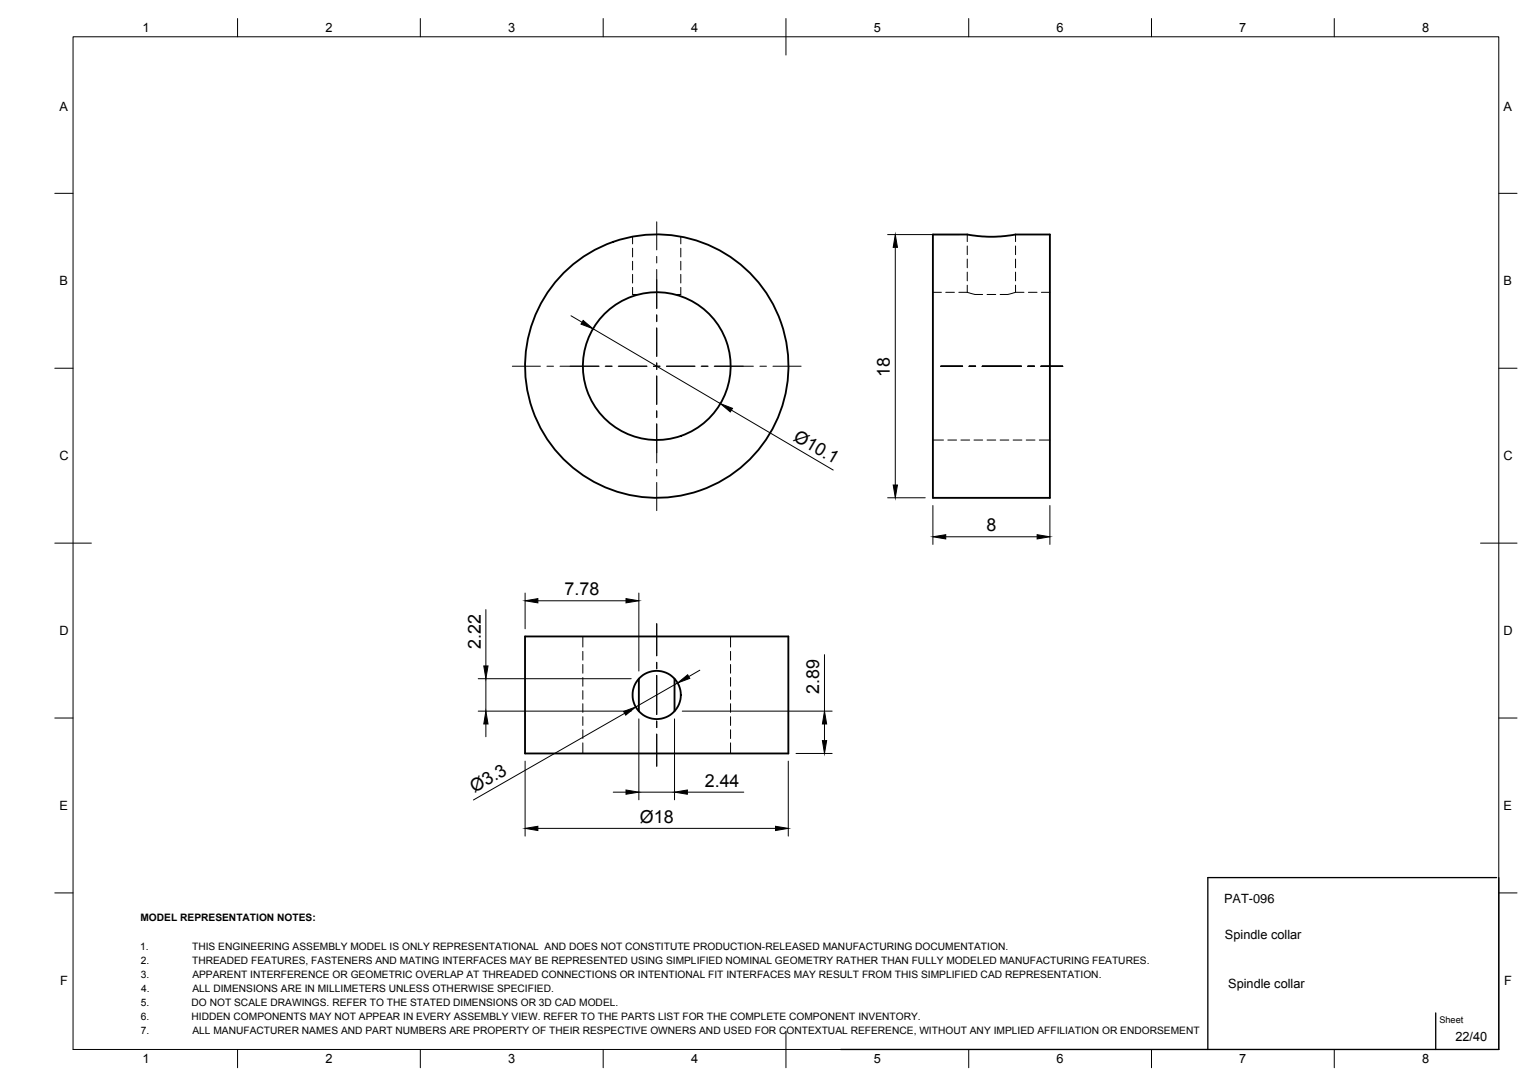
ISO-10303-21;
HEADER;
/* Generated by software containing ST-Developer
 * from STEP Tools, Inc. (www.steptools.com) 
 */

FILE_DESCRIPTION(
/* description */ ('PAT-096'),
/* implementation_level */ '2;1');

FILE_NAME(
/* name */ 'Spindle collar.step',
/* time_stamp */ '2026-10-29T17:03:14-07:00',
/* author */ (''),
/* organization */ (''),
/* preprocessor_version */ 'ST-DEVELOPER v20.2',
/* originating_system */ 'Autodesk Translation Framework v15.17.0.0',
/* authorisation */ '');

FILE_SCHEMA (('AUTOMOTIVE_DESIGN { 1 0 10303 214 3 1 1 }'));
ENDSEC;

DATA;
#10=MECHANICAL_DESIGN_GEOMETRIC_PRESENTATION_REPRESENTATION('',(#421),#10650);
#307=B_SPLINE_CURVE_WITH_KNOTS('',3,(#9836,#9837,#9838,#9839,#9840,#9841,
#9842,#9843,#9844,#9845,#9846,#9847,#9848,#9849),.UNSPECIFIED.,.F.,.F.,
(4,2,2,2,2,2,4),(0.618551524396293,0.626563103102765,0.689203386094988,
0.751843669087211,0.814483952079434,0.877124235071657,0.88513581377813),
 .UNSPECIFIED.);
#308=B_SPLINE_CURVE_WITH_KNOTS('',3,(#9853,#9854,#9855,#9856,#9857,#9858,
#9859,#9860),.UNSPECIFIED.,.F.,.F.,(4,2,2,4),(0.250614556362404,0.313254839354627,
0.37589512234685,0.383906701053323),.UNSPECIFIED.);
#309=B_SPLINE_CURVE_WITH_KNOTS('',3,(#9864,#9865,#9866,#9867,#9868,#9869,
#9870,#9871,#9872,#9873,#9874,#9875,#9876,#9877,#9878,#9879,#9880,#9881,
#9882,#9883,#9884,#9885,#9886,#9887,#9888,#9889),.UNSPECIFIED.,.F.,.F.,
(4,2,2,2,2,2,2,2,2,2,2,2,4),(0.,0.0623062782223143,0.124612556444629,0.186916384615149,
0.249220212785669,0.31152404095619,0.37382786912671,0.436134147349024,0.498440425571339,
0.560746703793653,0.623052982015967,0.685356810186488,0.747660638357008),
 .UNSPECIFIED.);
#310=B_SPLINE_CURVE_WITH_KNOTS('',3,(#9890,#9891,#9892,#9893,#9894,#9895,
#9896,#9897,#9898,#9899),.UNSPECIFIED.,.F.,.F.,(4,2,2,2,4),(0.747660638357008,
0.809964466527528,0.872268294698049,0.934574572920363,0.996880851142677),
 .UNSPECIFIED.);
#311=B_SPLINE_CURVE_WITH_KNOTS('',3,(#9900,#9901,#9902,#9903,#9904,#9905,
#9906,#9907),.UNSPECIFIED.,.F.,.F.,(4,2,2,4),(0.117322411671485,0.125333990377958,
0.187974273370181,0.250614556362404),.UNSPECIFIED.);
#351=SHAPE_REPRESENTATION_RELATIONSHIP('SRR','None',#10813,#382);
#382=ADVANCED_BREP_SHAPE_REPRESENTATION('',(#459),#10631);
#421=STYLED_ITEM('',(#11057),#459);
#459=MANIFOLD_SOLID_BREP('Body1',#5555);
#553=FACE_BOUND('',#1400,.T.);
#554=FACE_BOUND('',#1402,.T.);
#555=FACE_BOUND('',#1404,.T.);
#556=FACE_BOUND('',#1406,.T.);
#701=PLANE('',#6337);
#702=PLANE('',#6341);
#703=PLANE('',#6348);
#704=PLANE('',#6349);
#980=FACE_OUTER_BOUND('',#1396,.T.);
#981=FACE_OUTER_BOUND('',#1397,.T.);
#982=FACE_OUTER_BOUND('',#1398,.T.);
#983=FACE_OUTER_BOUND('',#1399,.T.);
#984=FACE_OUTER_BOUND('',#1401,.T.);
#985=FACE_OUTER_BOUND('',#1403,.T.);
#986=FACE_OUTER_BOUND('',#1405,.T.);
#1396=EDGE_LOOP('',(#4517,#4518));
#1397=EDGE_LOOP('',(#4519,#4520,#4521,#4522,#4523,#4524,#4525,#4526,#4527));
#1398=EDGE_LOOP('',(#4528,#4529));
#1399=EDGE_LOOP('',(#4530,#4531,#4532,#4533));
#1400=EDGE_LOOP('',(#4534,#4535,#4536,#4537,#4538));
#1401=EDGE_LOOP('',(#4539,#4540,#4541,#4542));
#1402=EDGE_LOOP('',(#4543,#4544));
#1403=EDGE_LOOP('',(#4545));
#1404=EDGE_LOOP('',(#4546));
#1405=EDGE_LOOP('',(#4547));
#1406=EDGE_LOOP('',(#4548));
#1769=LINE('',#9832,#2098);
#1770=LINE('',#9862,#2099);
#1771=LINE('',#9909,#2100);
#1772=LINE('',#9914,#2101);
#1773=LINE('',#9920,#2102);
#2098=VECTOR('',#7685,1.);
#2099=VECTOR('',#7692,0.165);
#2100=VECTOR('',#7695,1.);
#2101=VECTOR('',#7700,0.505);
#2102=VECTOR('',#7707,0.9);
#2466=CIRCLE('',#6338,0.165);
#2467=CIRCLE('',#6340,0.165);
#2468=CIRCLE('',#6343,0.505);
#2469=CIRCLE('',#6344,0.505);
#2470=CIRCLE('',#6346,0.9);
#2471=CIRCLE('',#6347,0.9);
#2853=VERTEX_POINT('',#9830);
#2854=VERTEX_POINT('',#9831);
#2855=VERTEX_POINT('',#9835);
#2856=VERTEX_POINT('',#9850);
#2857=VERTEX_POINT('',#9852);
#2858=VERTEX_POINT('',#9861);
#2859=VERTEX_POINT('',#9863);
#2860=VERTEX_POINT('',#9911);
#2861=VERTEX_POINT('',#9913);
#2862=VERTEX_POINT('',#9917);
#2863=VERTEX_POINT('',#9919);
#3437=EDGE_CURVE('',#2853,#2854,#1769,.T.);
#3438=EDGE_CURVE('',#2853,#2854,#2466,.T.);
#3439=EDGE_CURVE('',#2855,#2853,#307,.T.);
#3440=EDGE_CURVE('',#2856,#2855,#2467,.T.);
#3441=EDGE_CURVE('',#2857,#2856,#308,.T.);
#3442=EDGE_CURVE('',#2857,#2858,#1770,.T.);
#3443=EDGE_CURVE('',#2859,#2858,#309,.T.);
#3444=EDGE_CURVE('',#2858,#2859,#310,.T.);
#3445=EDGE_CURVE('',#2854,#2857,#311,.T.);
#3446=EDGE_CURVE('',#2856,#2855,#1771,.T.);
#3447=EDGE_CURVE('',#2860,#2860,#2468,.T.);
#3448=EDGE_CURVE('',#2860,#2861,#1772,.T.);
#3449=EDGE_CURVE('',#2861,#2861,#2469,.T.);
#3450=EDGE_CURVE('',#2862,#2862,#2470,.T.);
#3451=EDGE_CURVE('',#2862,#2863,#1773,.T.);
#3452=EDGE_CURVE('',#2863,#2863,#2471,.T.);
#4517=ORIENTED_EDGE('',*,*,#3437,.F.);
#4518=ORIENTED_EDGE('',*,*,#3438,.T.);
#4519=ORIENTED_EDGE('',*,*,#3439,.F.);
#4520=ORIENTED_EDGE('',*,*,#3440,.F.);
#4521=ORIENTED_EDGE('',*,*,#3441,.F.);
#4522=ORIENTED_EDGE('',*,*,#3442,.T.);
#4523=ORIENTED_EDGE('',*,*,#3443,.F.);
#4524=ORIENTED_EDGE('',*,*,#3444,.F.);
#4525=ORIENTED_EDGE('',*,*,#3442,.F.);
#4526=ORIENTED_EDGE('',*,*,#3445,.F.);
#4527=ORIENTED_EDGE('',*,*,#3438,.F.);
#4528=ORIENTED_EDGE('',*,*,#3446,.F.);
#4529=ORIENTED_EDGE('',*,*,#3440,.T.);
#4530=ORIENTED_EDGE('',*,*,#3447,.F.);
#4531=ORIENTED_EDGE('',*,*,#3448,.T.);
#4532=ORIENTED_EDGE('',*,*,#3449,.T.);
#4533=ORIENTED_EDGE('',*,*,#3448,.F.);
#4534=ORIENTED_EDGE('',*,*,#3445,.T.);
#4535=ORIENTED_EDGE('',*,*,#3441,.T.);
#4536=ORIENTED_EDGE('',*,*,#3446,.T.);
#4537=ORIENTED_EDGE('',*,*,#3439,.T.);
#4538=ORIENTED_EDGE('',*,*,#3437,.T.);
#4539=ORIENTED_EDGE('',*,*,#3450,.F.);
#4540=ORIENTED_EDGE('',*,*,#3451,.T.);
#4541=ORIENTED_EDGE('',*,*,#3452,.T.);
#4542=ORIENTED_EDGE('',*,*,#3451,.F.);
#4543=ORIENTED_EDGE('',*,*,#3443,.T.);
#4544=ORIENTED_EDGE('',*,*,#3444,.T.);
#4545=ORIENTED_EDGE('',*,*,#3450,.T.);
#4546=ORIENTED_EDGE('',*,*,#3447,.T.);
#4547=ORIENTED_EDGE('',*,*,#3452,.F.);
#4548=ORIENTED_EDGE('',*,*,#3449,.F.);
#5146=CYLINDRICAL_SURFACE('',#6339,0.165);
#5147=CYLINDRICAL_SURFACE('',#6342,0.505);
#5148=CYLINDRICAL_SURFACE('',#6345,0.9);
#5385=ADVANCED_FACE('',(#980),#701,.T.);
#5386=ADVANCED_FACE('',(#981),#5146,.F.);
#5387=ADVANCED_FACE('',(#982),#702,.T.);
#5388=ADVANCED_FACE('',(#983,#553),#5147,.F.);
#5389=ADVANCED_FACE('',(#984,#554),#5148,.T.);
#5390=ADVANCED_FACE('',(#985,#555),#703,.T.);
#5391=ADVANCED_FACE('',(#986,#556),#704,.F.);
#5555=CLOSED_SHELL('',(#5385,#5386,#5387,#5388,#5389,#5390,#5391));
#6336=AXIS2_PLACEMENT_3D('',#9828,#7681,#7682);
#6337=AXIS2_PLACEMENT_3D('',#9829,#7683,#7684);
#6338=AXIS2_PLACEMENT_3D('',#9833,#7686,#7687);
#6339=AXIS2_PLACEMENT_3D('',#9834,#7688,#7689);
#6340=AXIS2_PLACEMENT_3D('',#9851,#7690,#7691);
#6341=AXIS2_PLACEMENT_3D('',#9908,#7693,#7694);
#6342=AXIS2_PLACEMENT_3D('',#9910,#7696,#7697);
#6343=AXIS2_PLACEMENT_3D('',#9912,#7698,#7699);
#6344=AXIS2_PLACEMENT_3D('',#9915,#7701,#7702);
#6345=AXIS2_PLACEMENT_3D('',#9916,#7703,#7704);
#6346=AXIS2_PLACEMENT_3D('',#9918,#7705,#7706);
#6347=AXIS2_PLACEMENT_3D('',#9921,#7708,#7709);
#6348=AXIS2_PLACEMENT_3D('',#9922,#7710,#7711);
#6349=AXIS2_PLACEMENT_3D('',#9923,#7712,#7713);
#7681=DIRECTION('axis',(0.,0.,1.));
#7682=DIRECTION('refdir',(1.,0.,0.));
#7683=DIRECTION('center_axis',(1.,0.,0.));
#7684=DIRECTION('ref_axis',(0.,0.,-1.));
#7685=DIRECTION('',(0.,0.,1.));
#7686=DIRECTION('center_axis',(1.,0.,0.));
#7687=DIRECTION('ref_axis',(0.,0.,-1.));
#7688=DIRECTION('center_axis',(1.,0.,0.));
#7689=DIRECTION('ref_axis',(0.,0.,-1.));
#7690=DIRECTION('center_axis',(1.,0.,0.));
#7691=DIRECTION('ref_axis',(0.,0.,-1.));
#7692=DIRECTION('',(1.,0.,0.));
#7693=DIRECTION('center_axis',(1.,0.,0.));
#7694=DIRECTION('ref_axis',(0.,0.,-1.));
#7695=DIRECTION('',(0.,0.,-1.));
#7696=DIRECTION('center_axis',(0.,0.,1.));
#7697=DIRECTION('ref_axis',(1.,0.,0.));
#7698=DIRECTION('center_axis',(0.,0.,-1.));
#7699=DIRECTION('ref_axis',(1.,0.,0.));
#7700=DIRECTION('',(0.,0.,-1.));
#7701=DIRECTION('center_axis',(0.,0.,-1.));
#7702=DIRECTION('ref_axis',(1.,0.,0.));
#7703=DIRECTION('center_axis',(0.,0.,1.));
#7704=DIRECTION('ref_axis',(1.,0.,0.));
#7705=DIRECTION('center_axis',(0.,0.,1.));
#7706=DIRECTION('ref_axis',(1.,0.,0.));
#7707=DIRECTION('',(0.,0.,-1.));
#7708=DIRECTION('center_axis',(0.,0.,1.));
#7709=DIRECTION('ref_axis',(1.,0.,0.));
#7710=DIRECTION('center_axis',(0.,0.,1.));
#7711=DIRECTION('ref_axis',(1.,0.,0.));
#7712=DIRECTION('center_axis',(0.,0.,1.));
#7713=DIRECTION('ref_axis',(1.,0.,0.));
#9828=CARTESIAN_POINT('',(0.,0.,0.));
#9829=CARTESIAN_POINT('Origin',(0.49,0.,1.4));
#9830=CARTESIAN_POINT('',(0.49,0.122167917228706,1.28909463493591));
#9831=CARTESIAN_POINT('',(0.49,0.122167917228706,1.51090536506409));
#9832=CARTESIAN_POINT('',(0.49,0.122167917228706,1.));
#9833=CARTESIAN_POINT('Origin',(0.49,0.,1.4));
#9834=CARTESIAN_POINT('Origin',(0.49,0.,1.4));
#9835=CARTESIAN_POINT('',(0.49,-0.122167917228706,1.28909463493591));
#9836=CARTESIAN_POINT('Ctrl Pts',(0.49,-0.122167917228706,1.28909463493591));
#9837=CARTESIAN_POINT('Ctrl Pts',(0.490448531679987,-0.120368913626296,
1.28711294069536));
#9838=CARTESIAN_POINT('Ctrl Pts',(0.490895245371685,-0.118534896565231,
1.28518965877367));
#9839=CARTESIAN_POINT('Ctrl Pts',(0.494795015531646,-0.102111993019358,
1.2687667552278));
#9840=CARTESIAN_POINT('Ctrl Pts',(0.498442514607594,-0.0836597150224318,
1.25609154388858));
#9841=CARTESIAN_POINT('Ctrl Pts',(0.50357781976106,-0.0430495960471595,
1.23920409039234));
#9842=CARTESIAN_POINT('Ctrl Pts',(0.505,-0.020880094330741,1.235));
#9843=CARTESIAN_POINT('Ctrl Pts',(0.505,0.020880094330741,1.235));
#9844=CARTESIAN_POINT('Ctrl Pts',(0.50357781976106,0.0430495960471595,1.23920409039234));
#9845=CARTESIAN_POINT('Ctrl Pts',(0.498442514607594,0.0836597150224318,
1.25609154388858));
#9846=CARTESIAN_POINT('Ctrl Pts',(0.494795015531646,0.102111993019358,1.2687667552278));
#9847=CARTESIAN_POINT('Ctrl Pts',(0.490895245371684,0.118534896565231,1.28518965877367));
#9848=CARTESIAN_POINT('Ctrl Pts',(0.490448531679987,0.120368913626296,1.28711294069536));
#9849=CARTESIAN_POINT('Ctrl Pts',(0.49,0.122167917228706,1.28909463493591));
#9850=CARTESIAN_POINT('',(0.49,-0.122167917228706,1.51090536506409));
#9851=CARTESIAN_POINT('Origin',(0.49,0.,1.4));
#9852=CARTESIAN_POINT('',(0.505,-1.70422299968729E-17,1.565));
#9853=CARTESIAN_POINT('Ctrl Pts',(0.505,-6.93889390390723E-18,1.565));
#9854=CARTESIAN_POINT('Ctrl Pts',(0.505,-0.020880094330741,1.565));
#9855=CARTESIAN_POINT('Ctrl Pts',(0.50357781976106,-0.0430495960471595,
1.56079590960766));
#9856=CARTESIAN_POINT('Ctrl Pts',(0.498442514607594,-0.0836597150224318,
1.54390845611142));
#9857=CARTESIAN_POINT('Ctrl Pts',(0.494795015531646,-0.102111993019358,
1.5312332447722));
#9858=CARTESIAN_POINT('Ctrl Pts',(0.490895245371684,-0.118534896565231,
1.51481034122633));
#9859=CARTESIAN_POINT('Ctrl Pts',(0.490448531679987,-0.120368913626296,
1.51288705930464));
#9860=CARTESIAN_POINT('Ctrl Pts',(0.49,-0.122167917228706,1.51090536506409));
#9861=CARTESIAN_POINT('',(0.9,-2.02066721859313E-17,1.565));
#9862=CARTESIAN_POINT('',(0.49,-2.02066721859313E-17,1.565));
#9863=CARTESIAN_POINT('',(0.884745726183518,0.165,1.4));
#9864=CARTESIAN_POINT('Ctrl Pts',(0.884745726183518,0.165,1.4));
#9865=CARTESIAN_POINT('Ctrl Pts',(0.884745726183518,0.165,1.37923124059256));
#9866=CARTESIAN_POINT('Ctrl Pts',(0.885552759505264,0.160839719007584,1.35711110492666));
#9867=CARTESIAN_POINT('Ctrl Pts',(0.888448648150043,0.143986470216691,1.31647293736623));
#9868=CARTESIAN_POINT('Ctrl Pts',(0.890493604851638,0.131295993814186,1.29795075602263));
#9869=CARTESIAN_POINT('Ctrl Pts',(0.89431723432394,0.102049819008125,1.26870458121656));
#9870=CARTESIAN_POINT('Ctrl Pts',(0.896347088899543,0.0835273920906824,
1.25601365401642));
#9871=CARTESIAN_POINT('Ctrl Pts',(0.899208271860583,0.0428883760934127,
1.23916007816136));
#9872=CARTESIAN_POINT('Ctrl Pts',(0.9,0.0207679427235068,1.235));
#9873=CARTESIAN_POINT('Ctrl Pts',(0.9,-0.0207679427235068,1.235));
#9874=CARTESIAN_POINT('Ctrl Pts',(0.899208271860583,-0.0428883760934127,
1.23916007816136));
#9875=CARTESIAN_POINT('Ctrl Pts',(0.896347088899543,-0.0835273920906823,
1.25601365401642));
#9876=CARTESIAN_POINT('Ctrl Pts',(0.89431723432394,-0.102049819008125,1.26870458121656));
#9877=CARTESIAN_POINT('Ctrl Pts',(0.890493604851638,-0.131295993814186,
1.29795075602263));
#9878=CARTESIAN_POINT('Ctrl Pts',(0.888448648150043,-0.143986470216691,
1.31647293736623));
#9879=CARTESIAN_POINT('Ctrl Pts',(0.885552759505264,-0.160839719007584,
1.35711110492666));
#9880=CARTESIAN_POINT('Ctrl Pts',(0.884745726183518,-0.165,1.37923124059256));
#9881=CARTESIAN_POINT('Ctrl Pts',(0.884745726183518,-0.165,1.42076875940744));
#9882=CARTESIAN_POINT('Ctrl Pts',(0.885552759505264,-0.160839719007584,
1.44288889507334));
#9883=CARTESIAN_POINT('Ctrl Pts',(0.888448648150043,-0.14398647021669,1.48352706263377));
#9884=CARTESIAN_POINT('Ctrl Pts',(0.890493604851638,-0.131295993814186,
1.50204924397737));
#9885=CARTESIAN_POINT('Ctrl Pts',(0.89431723432394,-0.102049819008125,1.53129541878344));
#9886=CARTESIAN_POINT('Ctrl Pts',(0.896347088899543,-0.0835273920906824,
1.54398634598358));
#9887=CARTESIAN_POINT('Ctrl Pts',(0.899208271860583,-0.0428883760934128,
1.56083992183864));
#9888=CARTESIAN_POINT('Ctrl Pts',(0.9,-0.0207679427235068,1.565));
#9889=CARTESIAN_POINT('Ctrl Pts',(0.9,-6.93889390390723E-18,1.565));
#9890=CARTESIAN_POINT('Ctrl Pts',(0.9,-3.46944695195361E-17,1.565));
#9891=CARTESIAN_POINT('Ctrl Pts',(0.9,0.0207679427235068,1.565));
#9892=CARTESIAN_POINT('Ctrl Pts',(0.899208271860583,0.0428883760934127,
1.56083992183864));
#9893=CARTESIAN_POINT('Ctrl Pts',(0.896347088899543,0.0835273920906824,
1.54398634598358));
#9894=CARTESIAN_POINT('Ctrl Pts',(0.89431723432394,0.102049819008125,1.53129541878344));
#9895=CARTESIAN_POINT('Ctrl Pts',(0.890493604851638,0.131295993814186,1.50204924397737));
#9896=CARTESIAN_POINT('Ctrl Pts',(0.888448648150043,0.143986470216691,1.48352706263377));
#9897=CARTESIAN_POINT('Ctrl Pts',(0.885552759505264,0.160839719007584,1.44288889507334));
#9898=CARTESIAN_POINT('Ctrl Pts',(0.884745726183518,0.165,1.42076875940744));
#9899=CARTESIAN_POINT('Ctrl Pts',(0.884745726183518,0.165,1.4));
#9900=CARTESIAN_POINT('Ctrl Pts',(0.49,0.122167917228706,1.51090536506409));
#9901=CARTESIAN_POINT('Ctrl Pts',(0.490448531679987,0.120368913626296,1.51288705930464));
#9902=CARTESIAN_POINT('Ctrl Pts',(0.490895245371685,0.118534896565231,1.51481034122633));
#9903=CARTESIAN_POINT('Ctrl Pts',(0.494795015531646,0.102111993019358,1.5312332447722));
#9904=CARTESIAN_POINT('Ctrl Pts',(0.498442514607594,0.0836597150224318,
1.54390845611142));
#9905=CARTESIAN_POINT('Ctrl Pts',(0.50357781976106,0.0430495960471594,1.56079590960766));
#9906=CARTESIAN_POINT('Ctrl Pts',(0.505,0.020880094330741,1.565));
#9907=CARTESIAN_POINT('Ctrl Pts',(0.505,0.,1.565));
#9908=CARTESIAN_POINT('Origin',(0.49,0.,1.4));
#9909=CARTESIAN_POINT('',(0.49,-0.122167917228706,1.));
#9910=CARTESIAN_POINT('Origin',(0.,0.,1.));
#9911=CARTESIAN_POINT('',(-0.505,-6.18446633569413E-17,1.8));
#9912=CARTESIAN_POINT('Origin',(0.,0.,1.8));
#9913=CARTESIAN_POINT('',(-0.505,-6.18446633569413E-17,1.));
#9914=CARTESIAN_POINT('',(-0.505,-6.18446633569413E-17,1.));
#9915=CARTESIAN_POINT('Origin',(0.,0.,1.));
#9916=CARTESIAN_POINT('Origin',(0.,0.,1.));
#9917=CARTESIAN_POINT('',(-0.9,-1.10218211923262E-16,1.8));
#9918=CARTESIAN_POINT('Origin',(0.,0.,1.8));
#9919=CARTESIAN_POINT('',(-0.9,-1.10218211923262E-16,1.));
#9920=CARTESIAN_POINT('',(-0.9,-1.10218211923262E-16,1.));
#9921=CARTESIAN_POINT('Origin',(0.,0.,1.));
#9922=CARTESIAN_POINT('Origin',(0.,0.,1.8));
#9923=CARTESIAN_POINT('Origin',(0.,0.,1.));
#10592=UNCERTAINTY_MEASURE_WITH_UNIT(LENGTH_MEASURE(0.001),#10651,
'DISTANCE_ACCURACY_VALUE',
'Maximum model space distance between geometric entities at asserted c
onnectivities');
#10611=UNCERTAINTY_MEASURE_WITH_UNIT(LENGTH_MEASURE(0.001),#10651,
'DISTANCE_ACCURACY_VALUE',
'Maximum model space distance between geometric entities at asserted c
onnectivities');
#10631=(
GEOMETRIC_REPRESENTATION_CONTEXT(3)
GLOBAL_UNCERTAINTY_ASSIGNED_CONTEXT((#10592))
GLOBAL_UNIT_ASSIGNED_CONTEXT((#10651,#10653,#10654))
REPRESENTATION_CONTEXT('','3D')
);
#10650=(
GEOMETRIC_REPRESENTATION_CONTEXT(3)
GLOBAL_UNCERTAINTY_ASSIGNED_CONTEXT((#10611))
GLOBAL_UNIT_ASSIGNED_CONTEXT((#10651,#10653,#10654))
REPRESENTATION_CONTEXT('','3D')
);
#10651=(
LENGTH_UNIT()
NAMED_UNIT(*)
SI_UNIT(.CENTI.,.METRE.)
);
#10653=(
NAMED_UNIT(*)
PLANE_ANGLE_UNIT()
SI_UNIT($,.RADIAN.)
);
#10654=(
NAMED_UNIT(*)
SI_UNIT($,.STERADIAN.)
SOLID_ANGLE_UNIT()
);
#10674=SHAPE_DEFINITION_REPRESENTATION(#10717,#10813);
#10717=PRODUCT_DEFINITION_SHAPE('',$,#10852);
#10813=SHAPE_REPRESENTATION('',(#6336),#10631);
#10832=PRODUCT_DEFINITION_CONTEXT('part definition',#10948,'design');
#10852=PRODUCT_DEFINITION('Spindle collar','Spindle collar',#10890,#10832);
#10890=PRODUCT_DEFINITION_FORMATION('',$,#10969);
#10948=APPLICATION_CONTEXT(
'Core Data for Automotive Mechanical Design Process');
#10949=PRODUCT_CONTEXT('part definition',#10948,'mechanical');
#10969=PRODUCT('Spindle collar','Spindle collar','Spindle collar',(#10949));
#11051=COLOUR_RGB('Sky Blue',0.24,0.69,0.87);
#11052=FILL_AREA_STYLE_COLOUR('',#11051);
#11053=FILL_AREA_STYLE('',(#11052));
#11054=SURFACE_STYLE_FILL_AREA(#11053);
#11055=SURFACE_SIDE_STYLE('',(#11054));
#11056=SURFACE_STYLE_USAGE(.BOTH.,#11055);
#11057=PRESENTATION_STYLE_ASSIGNMENT((#11056));
ENDSEC;
END-ISO-10303-21;
